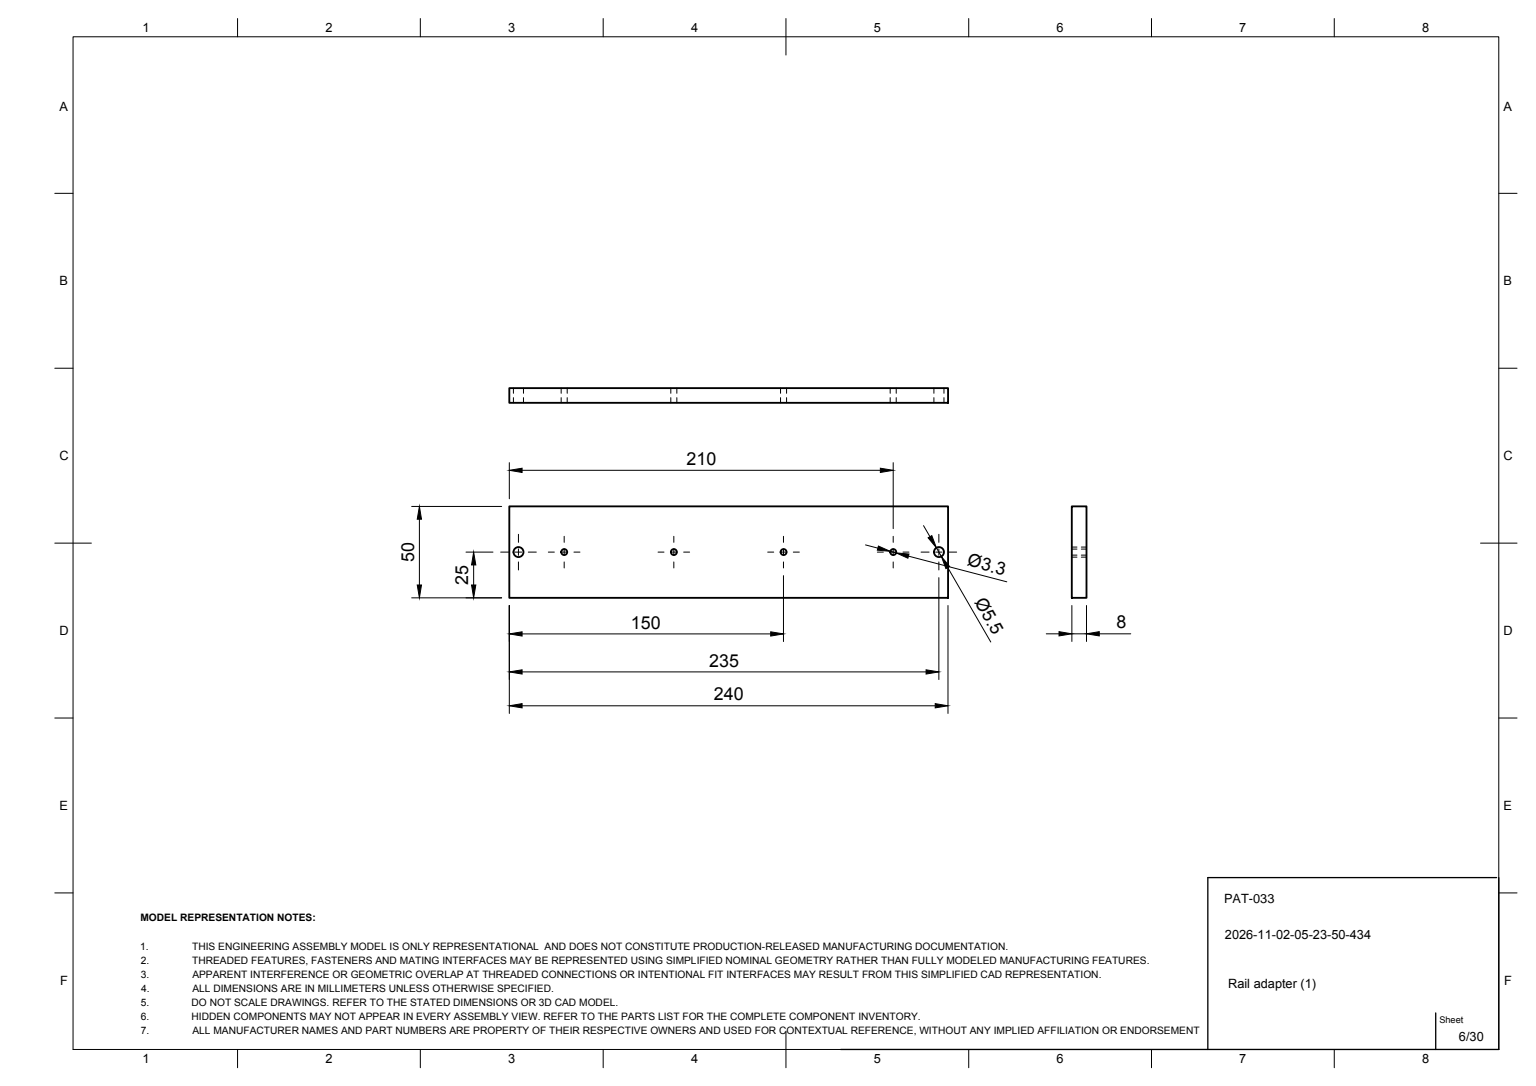
ISO-10303-21;
HEADER;
/* Generated by software containing ST-Developer
 * from STEP Tools, Inc. (www.steptools.com) 
 */

FILE_DESCRIPTION(
/* description */ ('Dual-rail gantry carriage'),
/* implementation_level */ '2;1');

FILE_NAME(
/* name */ 'Rail adapter (1).step',
/* time_stamp */ '2026-10-27T10:49:15-07:00',
/* author */ (''),
/* organization */ (''),
/* preprocessor_version */ 'ST-DEVELOPER v20.2',
/* originating_system */ 'Autodesk Translation Framework v15.17.0.0',
/* authorisation */ '');

FILE_SCHEMA (('AUTOMOTIVE_DESIGN { 1 0 10303 214 3 1 1 }'));
ENDSEC;

DATA;
#10=MECHANICAL_DESIGN_GEOMETRIC_PRESENTATION_REPRESENTATION('',(#586),#12804);
#524=SHAPE_REPRESENTATION_RELATIONSHIP('SRR','None',#13002,#555);
#555=ADVANCED_BREP_SHAPE_REPRESENTATION('',(#617),#12772);
#586=STYLED_ITEM('',(#13240),#617);
#617=MANIFOLD_SOLID_BREP('Body1',#7364);
#654=FACE_BOUND('',#1472,.T.);
#655=FACE_BOUND('',#1473,.T.);
#656=FACE_BOUND('',#1474,.T.);
#657=FACE_BOUND('',#1475,.T.);
#658=FACE_BOUND('',#1476,.T.);
#659=FACE_BOUND('',#1477,.T.);
#660=FACE_BOUND('',#1479,.T.);
#661=FACE_BOUND('',#1480,.T.);
#662=FACE_BOUND('',#1481,.T.);
#663=FACE_BOUND('',#1482,.T.);
#664=FACE_BOUND('',#1483,.T.);
#665=FACE_BOUND('',#1484,.T.);
#770=PLANE('',#7787);
#771=PLANE('',#7788);
#772=PLANE('',#7789);
#773=PLANE('',#7790);
#774=PLANE('',#7791);
#775=PLANE('',#7792);
#1060=FACE_OUTER_BOUND('',#1461,.T.);
#1061=FACE_OUTER_BOUND('',#1462,.T.);
#1062=FACE_OUTER_BOUND('',#1463,.T.);
#1063=FACE_OUTER_BOUND('',#1464,.T.);
#1064=FACE_OUTER_BOUND('',#1465,.T.);
#1065=FACE_OUTER_BOUND('',#1466,.T.);
#1066=FACE_OUTER_BOUND('',#1467,.T.);
#1067=FACE_OUTER_BOUND('',#1468,.T.);
#1068=FACE_OUTER_BOUND('',#1469,.T.);
#1069=FACE_OUTER_BOUND('',#1470,.T.);
#1070=FACE_OUTER_BOUND('',#1471,.T.);
#1071=FACE_OUTER_BOUND('',#1478,.T.);
#1461=EDGE_LOOP('',(#5127,#5128,#5129,#5130));
#1462=EDGE_LOOP('',(#5131,#5132,#5133,#5134));
#1463=EDGE_LOOP('',(#5135,#5136,#5137,#5138));
#1464=EDGE_LOOP('',(#5139,#5140,#5141,#5142));
#1465=EDGE_LOOP('',(#5143,#5144,#5145,#5146));
#1466=EDGE_LOOP('',(#5147,#5148,#5149,#5150));
#1467=EDGE_LOOP('',(#5151,#5152,#5153,#5154));
#1468=EDGE_LOOP('',(#5155,#5156,#5157,#5158));
#1469=EDGE_LOOP('',(#5159,#5160,#5161,#5162));
#1470=EDGE_LOOP('',(#5163,#5164,#5165,#5166));
#1471=EDGE_LOOP('',(#5167,#5168,#5169,#5170));
#1472=EDGE_LOOP('',(#5171));
#1473=EDGE_LOOP('',(#5172));
#1474=EDGE_LOOP('',(#5173));
#1475=EDGE_LOOP('',(#5174));
#1476=EDGE_LOOP('',(#5175));
#1477=EDGE_LOOP('',(#5176));
#1478=EDGE_LOOP('',(#5177,#5178,#5179,#5180));
#1479=EDGE_LOOP('',(#5181));
#1480=EDGE_LOOP('',(#5182));
#1481=EDGE_LOOP('',(#5183));
#1482=EDGE_LOOP('',(#5184));
#1483=EDGE_LOOP('',(#5185));
#1484=EDGE_LOOP('',(#5186));
#1966=LINE('',#10758,#2675);
#1967=LINE('',#10764,#2676);
#1968=LINE('',#10770,#2677);
#1969=LINE('',#10776,#2678);
#1970=LINE('',#10782,#2679);
#1971=LINE('',#10788,#2680);
#1972=LINE('',#10793,#2681);
#1973=LINE('',#10795,#2682);
#1974=LINE('',#10797,#2683);
#1975=LINE('',#10798,#2684);
#1976=LINE('',#10801,#2685);
#1977=LINE('',#10803,#2686);
#1978=LINE('',#10804,#2687);
#1979=LINE('',#10807,#2688);
#1980=LINE('',#10809,#2689);
#1981=LINE('',#10810,#2690);
#1982=LINE('',#10812,#2691);
#1983=LINE('',#10813,#2692);
#2675=VECTOR('',#8565,0.164999999999999);
#2676=VECTOR('',#8572,0.164999999999999);
#2677=VECTOR('',#8579,0.164999999999999);
#2678=VECTOR('',#8586,0.164999999999999);
#2679=VECTOR('',#8593,0.275);
#2680=VECTOR('',#8600,0.274999999999999);
#2681=VECTOR('',#8605,1.);
#2682=VECTOR('',#8606,1.);
#2683=VECTOR('',#8607,1.);
#2684=VECTOR('',#8608,1.);
#2685=VECTOR('',#8611,1.);
#2686=VECTOR('',#8612,1.);
#2687=VECTOR('',#8613,1.);
#2688=VECTOR('',#8616,1.);
#2689=VECTOR('',#8617,1.);
#2690=VECTOR('',#8618,1.);
#2691=VECTOR('',#8621,1.);
#2692=VECTOR('',#8622,1.);
#3378=CIRCLE('',#7770,0.164999999999999);
#3379=CIRCLE('',#7771,0.164999999999999);
#3380=CIRCLE('',#7773,0.164999999999999);
#3381=CIRCLE('',#7774,0.164999999999999);
#3382=CIRCLE('',#7776,0.164999999999999);
#3383=CIRCLE('',#7777,0.164999999999999);
#3384=CIRCLE('',#7779,0.164999999999999);
#3385=CIRCLE('',#7780,0.164999999999999);
#3386=CIRCLE('',#7782,0.275);
#3387=CIRCLE('',#7783,0.275);
#3388=CIRCLE('',#7785,0.274999999999999);
#3389=CIRCLE('',#7786,0.274999999999999);
#3586=VERTEX_POINT('',#10755);
#3587=VERTEX_POINT('',#10757);
#3588=VERTEX_POINT('',#10761);
#3589=VERTEX_POINT('',#10763);
#3590=VERTEX_POINT('',#10767);
#3591=VERTEX_POINT('',#10769);
#3592=VERTEX_POINT('',#10773);
#3593=VERTEX_POINT('',#10775);
#3594=VERTEX_POINT('',#10779);
#3595=VERTEX_POINT('',#10781);
#3596=VERTEX_POINT('',#10785);
#3597=VERTEX_POINT('',#10787);
#3598=VERTEX_POINT('',#10791);
#3599=VERTEX_POINT('',#10792);
#3600=VERTEX_POINT('',#10794);
#3601=VERTEX_POINT('',#10796);
#3602=VERTEX_POINT('',#10800);
#3603=VERTEX_POINT('',#10802);
#3604=VERTEX_POINT('',#10806);
#3605=VERTEX_POINT('',#10808);
#4186=EDGE_CURVE('',#3586,#3586,#3378,.T.);
#4187=EDGE_CURVE('',#3586,#3587,#1966,.T.);
#4188=EDGE_CURVE('',#3587,#3587,#3379,.T.);
#4189=EDGE_CURVE('',#3588,#3588,#3380,.T.);
#4190=EDGE_CURVE('',#3588,#3589,#1967,.T.);
#4191=EDGE_CURVE('',#3589,#3589,#3381,.T.);
#4192=EDGE_CURVE('',#3590,#3590,#3382,.T.);
#4193=EDGE_CURVE('',#3590,#3591,#1968,.T.);
#4194=EDGE_CURVE('',#3591,#3591,#3383,.T.);
#4195=EDGE_CURVE('',#3592,#3592,#3384,.T.);
#4196=EDGE_CURVE('',#3592,#3593,#1969,.T.);
#4197=EDGE_CURVE('',#3593,#3593,#3385,.T.);
#4198=EDGE_CURVE('',#3594,#3594,#3386,.T.);
#4199=EDGE_CURVE('',#3594,#3595,#1970,.T.);
#4200=EDGE_CURVE('',#3595,#3595,#3387,.T.);
#4201=EDGE_CURVE('',#3596,#3596,#3388,.T.);
#4202=EDGE_CURVE('',#3596,#3597,#1971,.T.);
#4203=EDGE_CURVE('',#3597,#3597,#3389,.T.);
#4204=EDGE_CURVE('',#3598,#3599,#1972,.T.);
#4205=EDGE_CURVE('',#3599,#3600,#1973,.T.);
#4206=EDGE_CURVE('',#3601,#3600,#1974,.T.);
#4207=EDGE_CURVE('',#3598,#3601,#1975,.T.);
#4208=EDGE_CURVE('',#3602,#3598,#1976,.T.);
#4209=EDGE_CURVE('',#3603,#3601,#1977,.T.);
#4210=EDGE_CURVE('',#3602,#3603,#1978,.T.);
#4211=EDGE_CURVE('',#3604,#3602,#1979,.T.);
#4212=EDGE_CURVE('',#3605,#3603,#1980,.T.);
#4213=EDGE_CURVE('',#3604,#3605,#1981,.T.);
#4214=EDGE_CURVE('',#3599,#3604,#1982,.T.);
#4215=EDGE_CURVE('',#3600,#3605,#1983,.T.);
#5127=ORIENTED_EDGE('',*,*,#4186,.F.);
#5128=ORIENTED_EDGE('',*,*,#4187,.T.);
#5129=ORIENTED_EDGE('',*,*,#4188,.F.);
#5130=ORIENTED_EDGE('',*,*,#4187,.F.);
#5131=ORIENTED_EDGE('',*,*,#4189,.F.);
#5132=ORIENTED_EDGE('',*,*,#4190,.T.);
#5133=ORIENTED_EDGE('',*,*,#4191,.F.);
#5134=ORIENTED_EDGE('',*,*,#4190,.F.);
#5135=ORIENTED_EDGE('',*,*,#4192,.F.);
#5136=ORIENTED_EDGE('',*,*,#4193,.T.);
#5137=ORIENTED_EDGE('',*,*,#4194,.F.);
#5138=ORIENTED_EDGE('',*,*,#4193,.F.);
#5139=ORIENTED_EDGE('',*,*,#4195,.F.);
#5140=ORIENTED_EDGE('',*,*,#4196,.T.);
#5141=ORIENTED_EDGE('',*,*,#4197,.F.);
#5142=ORIENTED_EDGE('',*,*,#4196,.F.);
#5143=ORIENTED_EDGE('',*,*,#4198,.F.);
#5144=ORIENTED_EDGE('',*,*,#4199,.T.);
#5145=ORIENTED_EDGE('',*,*,#4200,.F.);
#5146=ORIENTED_EDGE('',*,*,#4199,.F.);
#5147=ORIENTED_EDGE('',*,*,#4201,.F.);
#5148=ORIENTED_EDGE('',*,*,#4202,.T.);
#5149=ORIENTED_EDGE('',*,*,#4203,.F.);
#5150=ORIENTED_EDGE('',*,*,#4202,.F.);
#5151=ORIENTED_EDGE('',*,*,#4204,.T.);
#5152=ORIENTED_EDGE('',*,*,#4205,.T.);
#5153=ORIENTED_EDGE('',*,*,#4206,.F.);
#5154=ORIENTED_EDGE('',*,*,#4207,.F.);
#5155=ORIENTED_EDGE('',*,*,#4208,.T.);
#5156=ORIENTED_EDGE('',*,*,#4207,.T.);
#5157=ORIENTED_EDGE('',*,*,#4209,.F.);
#5158=ORIENTED_EDGE('',*,*,#4210,.F.);
#5159=ORIENTED_EDGE('',*,*,#4211,.T.);
#5160=ORIENTED_EDGE('',*,*,#4210,.T.);
#5161=ORIENTED_EDGE('',*,*,#4212,.F.);
#5162=ORIENTED_EDGE('',*,*,#4213,.F.);
#5163=ORIENTED_EDGE('',*,*,#4214,.T.);
#5164=ORIENTED_EDGE('',*,*,#4213,.T.);
#5165=ORIENTED_EDGE('',*,*,#4215,.F.);
#5166=ORIENTED_EDGE('',*,*,#4205,.F.);
#5167=ORIENTED_EDGE('',*,*,#4215,.T.);
#5168=ORIENTED_EDGE('',*,*,#4212,.T.);
#5169=ORIENTED_EDGE('',*,*,#4209,.T.);
#5170=ORIENTED_EDGE('',*,*,#4206,.T.);
#5171=ORIENTED_EDGE('',*,*,#4203,.T.);
#5172=ORIENTED_EDGE('',*,*,#4200,.T.);
#5173=ORIENTED_EDGE('',*,*,#4197,.T.);
#5174=ORIENTED_EDGE('',*,*,#4194,.T.);
#5175=ORIENTED_EDGE('',*,*,#4191,.T.);
#5176=ORIENTED_EDGE('',*,*,#4188,.T.);
#5177=ORIENTED_EDGE('',*,*,#4214,.F.);
#5178=ORIENTED_EDGE('',*,*,#4204,.F.);
#5179=ORIENTED_EDGE('',*,*,#4208,.F.);
#5180=ORIENTED_EDGE('',*,*,#4211,.F.);
#5181=ORIENTED_EDGE('',*,*,#4201,.T.);
#5182=ORIENTED_EDGE('',*,*,#4198,.T.);
#5183=ORIENTED_EDGE('',*,*,#4195,.T.);
#5184=ORIENTED_EDGE('',*,*,#4192,.T.);
#5185=ORIENTED_EDGE('',*,*,#4189,.T.);
#5186=ORIENTED_EDGE('',*,*,#4186,.T.);
#6895=CYLINDRICAL_SURFACE('',#7769,0.164999999999999);
#6896=CYLINDRICAL_SURFACE('',#7772,0.164999999999999);
#6897=CYLINDRICAL_SURFACE('',#7775,0.164999999999999);
#6898=CYLINDRICAL_SURFACE('',#7778,0.164999999999999);
#6899=CYLINDRICAL_SURFACE('',#7781,0.275);
#6900=CYLINDRICAL_SURFACE('',#7784,0.274999999999999);
#6986=ADVANCED_FACE('',(#1060),#6895,.F.);
#6987=ADVANCED_FACE('',(#1061),#6896,.F.);
#6988=ADVANCED_FACE('',(#1062),#6897,.F.);
#6989=ADVANCED_FACE('',(#1063),#6898,.F.);
#6990=ADVANCED_FACE('',(#1064),#6899,.F.);
#6991=ADVANCED_FACE('',(#1065),#6900,.F.);
#6992=ADVANCED_FACE('',(#1066),#770,.T.);
#6993=ADVANCED_FACE('',(#1067),#771,.T.);
#6994=ADVANCED_FACE('',(#1068),#772,.T.);
#6995=ADVANCED_FACE('',(#1069),#773,.T.);
#6996=ADVANCED_FACE('',(#1070,#654,#655,#656,#657,#658,#659),#774,.T.);
#6997=ADVANCED_FACE('',(#1071,#660,#661,#662,#663,#664,#665),#775,.F.);
#7364=CLOSED_SHELL('',(#6986,#6987,#6988,#6989,#6990,#6991,#6992,#6993,
#6994,#6995,#6996,#6997));
#7768=AXIS2_PLACEMENT_3D('',#10753,#8559,#8560);
#7769=AXIS2_PLACEMENT_3D('',#10754,#8561,#8562);
#7770=AXIS2_PLACEMENT_3D('',#10756,#8563,#8564);
#7771=AXIS2_PLACEMENT_3D('',#10759,#8566,#8567);
#7772=AXIS2_PLACEMENT_3D('',#10760,#8568,#8569);
#7773=AXIS2_PLACEMENT_3D('',#10762,#8570,#8571);
#7774=AXIS2_PLACEMENT_3D('',#10765,#8573,#8574);
#7775=AXIS2_PLACEMENT_3D('',#10766,#8575,#8576);
#7776=AXIS2_PLACEMENT_3D('',#10768,#8577,#8578);
#7777=AXIS2_PLACEMENT_3D('',#10771,#8580,#8581);
#7778=AXIS2_PLACEMENT_3D('',#10772,#8582,#8583);
#7779=AXIS2_PLACEMENT_3D('',#10774,#8584,#8585);
#7780=AXIS2_PLACEMENT_3D('',#10777,#8587,#8588);
#7781=AXIS2_PLACEMENT_3D('',#10778,#8589,#8590);
#7782=AXIS2_PLACEMENT_3D('',#10780,#8591,#8592);
#7783=AXIS2_PLACEMENT_3D('',#10783,#8594,#8595);
#7784=AXIS2_PLACEMENT_3D('',#10784,#8596,#8597);
#7785=AXIS2_PLACEMENT_3D('',#10786,#8598,#8599);
#7786=AXIS2_PLACEMENT_3D('',#10789,#8601,#8602);
#7787=AXIS2_PLACEMENT_3D('',#10790,#8603,#8604);
#7788=AXIS2_PLACEMENT_3D('',#10799,#8609,#8610);
#7789=AXIS2_PLACEMENT_3D('',#10805,#8614,#8615);
#7790=AXIS2_PLACEMENT_3D('',#10811,#8619,#8620);
#7791=AXIS2_PLACEMENT_3D('',#10814,#8623,#8624);
#7792=AXIS2_PLACEMENT_3D('',#10815,#8625,#8626);
#8559=DIRECTION('axis',(0.,0.,1.));
#8560=DIRECTION('refdir',(1.,0.,0.));
#8561=DIRECTION('center_axis',(0.,0.,1.));
#8562=DIRECTION('ref_axis',(1.,0.,0.));
#8563=DIRECTION('center_axis',(0.,0.,1.));
#8564=DIRECTION('ref_axis',(1.,0.,0.));
#8565=DIRECTION('',(0.,0.,1.));
#8566=DIRECTION('center_axis',(0.,0.,-1.));
#8567=DIRECTION('ref_axis',(1.,0.,0.));
#8568=DIRECTION('center_axis',(0.,0.,1.));
#8569=DIRECTION('ref_axis',(1.,0.,0.));
#8570=DIRECTION('center_axis',(0.,0.,1.));
#8571=DIRECTION('ref_axis',(1.,0.,0.));
#8572=DIRECTION('',(0.,0.,1.));
#8573=DIRECTION('center_axis',(0.,0.,-1.));
#8574=DIRECTION('ref_axis',(1.,0.,0.));
#8575=DIRECTION('center_axis',(0.,0.,1.));
#8576=DIRECTION('ref_axis',(1.,0.,0.));
#8577=DIRECTION('center_axis',(0.,0.,1.));
#8578=DIRECTION('ref_axis',(1.,0.,0.));
#8579=DIRECTION('',(0.,0.,1.));
#8580=DIRECTION('center_axis',(0.,0.,-1.));
#8581=DIRECTION('ref_axis',(1.,0.,0.));
#8582=DIRECTION('center_axis',(0.,0.,1.));
#8583=DIRECTION('ref_axis',(1.,0.,0.));
#8584=DIRECTION('center_axis',(0.,0.,1.));
#8585=DIRECTION('ref_axis',(1.,0.,0.));
#8586=DIRECTION('',(0.,0.,1.));
#8587=DIRECTION('center_axis',(0.,0.,-1.));
#8588=DIRECTION('ref_axis',(1.,0.,0.));
#8589=DIRECTION('center_axis',(0.,0.,1.));
#8590=DIRECTION('ref_axis',(1.,0.,0.));
#8591=DIRECTION('center_axis',(0.,0.,1.));
#8592=DIRECTION('ref_axis',(1.,0.,0.));
#8593=DIRECTION('',(0.,0.,1.));
#8594=DIRECTION('center_axis',(0.,0.,-1.));
#8595=DIRECTION('ref_axis',(1.,0.,0.));
#8596=DIRECTION('center_axis',(0.,0.,1.));
#8597=DIRECTION('ref_axis',(1.,0.,0.));
#8598=DIRECTION('center_axis',(0.,0.,1.));
#8599=DIRECTION('ref_axis',(1.,0.,0.));
#8600=DIRECTION('',(0.,0.,1.));
#8601=DIRECTION('center_axis',(0.,0.,-1.));
#8602=DIRECTION('ref_axis',(1.,0.,0.));
#8603=DIRECTION('center_axis',(0.,1.,0.));
#8604=DIRECTION('ref_axis',(-1.,0.,0.));
#8605=DIRECTION('',(-1.,0.,0.));
#8606=DIRECTION('',(0.,0.,1.));
#8607=DIRECTION('',(-1.,0.,0.));
#8608=DIRECTION('',(0.,0.,1.));
#8609=DIRECTION('center_axis',(1.,0.,0.));
#8610=DIRECTION('ref_axis',(0.,1.,0.));
#8611=DIRECTION('',(0.,1.,0.));
#8612=DIRECTION('',(0.,1.,0.));
#8613=DIRECTION('',(0.,0.,1.));
#8614=DIRECTION('center_axis',(0.,-1.,0.));
#8615=DIRECTION('ref_axis',(1.,0.,0.));
#8616=DIRECTION('',(1.,0.,0.));
#8617=DIRECTION('',(1.,0.,0.));
#8618=DIRECTION('',(0.,0.,1.));
#8619=DIRECTION('center_axis',(-1.,0.,0.));
#8620=DIRECTION('ref_axis',(0.,-1.,0.));
#8621=DIRECTION('',(0.,-1.,0.));
#8622=DIRECTION('',(0.,-1.,0.));
#8623=DIRECTION('center_axis',(0.,0.,1.));
#8624=DIRECTION('ref_axis',(1.,0.,0.));
#8625=DIRECTION('center_axis',(0.,0.,1.));
#8626=DIRECTION('ref_axis',(1.,0.,0.));
#10753=CARTESIAN_POINT('',(0.,0.,0.));
#10754=CARTESIAN_POINT('Origin',(23.,10.,1.9));
#10755=CARTESIAN_POINT('',(22.835,10.,2.));
#10756=CARTESIAN_POINT('Origin',(23.,10.,2.));
#10757=CARTESIAN_POINT('',(22.835,10.,2.8));
#10758=CARTESIAN_POINT('',(22.835,10.,1.9));
#10759=CARTESIAN_POINT('Origin',(23.,10.,2.8));
#10760=CARTESIAN_POINT('Origin',(17.,10.,1.9));
#10761=CARTESIAN_POINT('',(16.835,10.,2.));
#10762=CARTESIAN_POINT('Origin',(17.,10.,2.));
#10763=CARTESIAN_POINT('',(16.835,10.,2.8));
#10764=CARTESIAN_POINT('',(16.835,10.,1.9));
#10765=CARTESIAN_POINT('Origin',(17.,10.,2.8));
#10766=CARTESIAN_POINT('Origin',(11.,10.,1.9));
#10767=CARTESIAN_POINT('',(10.835,10.,2.));
#10768=CARTESIAN_POINT('Origin',(11.,10.,2.));
#10769=CARTESIAN_POINT('',(10.835,10.,2.8));
#10770=CARTESIAN_POINT('',(10.835,10.,1.9));
#10771=CARTESIAN_POINT('Origin',(11.,10.,2.8));
#10772=CARTESIAN_POINT('Origin',(29.,10.,1.9));
#10773=CARTESIAN_POINT('',(28.835,10.,2.));
#10774=CARTESIAN_POINT('Origin',(29.,10.,2.));
#10775=CARTESIAN_POINT('',(28.835,10.,2.8));
#10776=CARTESIAN_POINT('',(28.835,10.,1.9));
#10777=CARTESIAN_POINT('Origin',(29.,10.,2.8));
#10778=CARTESIAN_POINT('Origin',(8.5,10.,1.9));
#10779=CARTESIAN_POINT('',(8.225,10.,2.));
#10780=CARTESIAN_POINT('Origin',(8.5,10.,2.));
#10781=CARTESIAN_POINT('',(8.225,10.,2.8));
#10782=CARTESIAN_POINT('',(8.225,10.,1.9));
#10783=CARTESIAN_POINT('Origin',(8.5,10.,2.8));
#10784=CARTESIAN_POINT('Origin',(31.5,10.,1.9));
#10785=CARTESIAN_POINT('',(31.225,10.,2.));
#10786=CARTESIAN_POINT('Origin',(31.5,10.,2.));
#10787=CARTESIAN_POINT('',(31.225,10.,2.8));
#10788=CARTESIAN_POINT('',(31.225,10.,1.9));
#10789=CARTESIAN_POINT('Origin',(31.5,10.,2.8));
#10790=CARTESIAN_POINT('Origin',(32.,12.5,2.));
#10791=CARTESIAN_POINT('',(32.,12.5,2.));
#10792=CARTESIAN_POINT('',(8.,12.5,2.));
#10793=CARTESIAN_POINT('',(32.,12.5,2.));
#10794=CARTESIAN_POINT('',(8.,12.5,2.8));
#10795=CARTESIAN_POINT('',(8.,12.5,2.));
#10796=CARTESIAN_POINT('',(32.,12.5,2.8));
#10797=CARTESIAN_POINT('',(32.,12.5,2.8));
#10798=CARTESIAN_POINT('',(32.,12.5,2.));
#10799=CARTESIAN_POINT('Origin',(32.,7.5,2.));
#10800=CARTESIAN_POINT('',(32.,7.5,2.));
#10801=CARTESIAN_POINT('',(32.,7.5,2.));
#10802=CARTESIAN_POINT('',(32.,7.5,2.8));
#10803=CARTESIAN_POINT('',(32.,7.5,2.8));
#10804=CARTESIAN_POINT('',(32.,7.5,2.));
#10805=CARTESIAN_POINT('Origin',(8.,7.5,2.));
#10806=CARTESIAN_POINT('',(8.,7.5,2.));
#10807=CARTESIAN_POINT('',(8.,7.5,2.));
#10808=CARTESIAN_POINT('',(8.,7.5,2.8));
#10809=CARTESIAN_POINT('',(8.,7.5,2.8));
#10810=CARTESIAN_POINT('',(8.,7.5,2.));
#10811=CARTESIAN_POINT('Origin',(8.,12.5,2.));
#10812=CARTESIAN_POINT('',(8.,12.5,2.));
#10813=CARTESIAN_POINT('',(8.,12.5,2.8));
#10814=CARTESIAN_POINT('Origin',(20.,10.,2.8));
#10815=CARTESIAN_POINT('Origin',(20.,10.,2.));
#12736=UNCERTAINTY_MEASURE_WITH_UNIT(LENGTH_MEASURE(0.001),#12805,
'DISTANCE_ACCURACY_VALUE',
'Maximum model space distance between geometric entities at asserted c
onnectivities');
#12768=UNCERTAINTY_MEASURE_WITH_UNIT(LENGTH_MEASURE(0.001),#12805,
'DISTANCE_ACCURACY_VALUE',
'Maximum model space distance between geometric entities at asserted c
onnectivities');
#12772=(
GEOMETRIC_REPRESENTATION_CONTEXT(3)
GLOBAL_UNCERTAINTY_ASSIGNED_CONTEXT((#12736))
GLOBAL_UNIT_ASSIGNED_CONTEXT((#12805,#12807,#12808))
REPRESENTATION_CONTEXT('','3D')
);
#12804=(
GEOMETRIC_REPRESENTATION_CONTEXT(3)
GLOBAL_UNCERTAINTY_ASSIGNED_CONTEXT((#12768))
GLOBAL_UNIT_ASSIGNED_CONTEXT((#12805,#12807,#12808))
REPRESENTATION_CONTEXT('','3D')
);
#12805=(
LENGTH_UNIT()
NAMED_UNIT(*)
SI_UNIT(.CENTI.,.METRE.)
);
#12807=(
NAMED_UNIT(*)
PLANE_ANGLE_UNIT()
SI_UNIT($,.RADIAN.)
);
#12808=(
NAMED_UNIT(*)
SI_UNIT($,.STERADIAN.)
SOLID_ANGLE_UNIT()
);
#12812=SHAPE_DEFINITION_REPRESENTATION(#12847,#13002);
#12847=PRODUCT_DEFINITION_SHAPE('',$,#13038);
#13002=SHAPE_REPRESENTATION('',(#7768),#12772);
#13034=PRODUCT_DEFINITION_CONTEXT('part definition',#13141,'design');
#13038=PRODUCT_DEFINITION('Rail adapter (1)','Rail adapter (1)',#13073,#13034);
#13073=PRODUCT_DEFINITION_FORMATION('',$,#13146);
#13141=APPLICATION_CONTEXT(
'Core Data for Automotive Mechanical Design Process');
#13142=PRODUCT_CONTEXT('part definition',#13141,'mechanical');
#13146=PRODUCT('Rail adapter (1)','Rail adapter (1)','Rail adapter (1)',(#13142));
#13234=COLOUR_RGB('Sky Blue',0.24,0.69,0.87);
#13235=FILL_AREA_STYLE_COLOUR('',#13234);
#13236=FILL_AREA_STYLE('',(#13235));
#13237=SURFACE_STYLE_FILL_AREA(#13236);
#13238=SURFACE_SIDE_STYLE('',(#13237));
#13239=SURFACE_STYLE_USAGE(.BOTH.,#13238);
#13240=PRESENTATION_STYLE_ASSIGNMENT((#13239));
ENDSEC;
END-ISO-10303-21;
